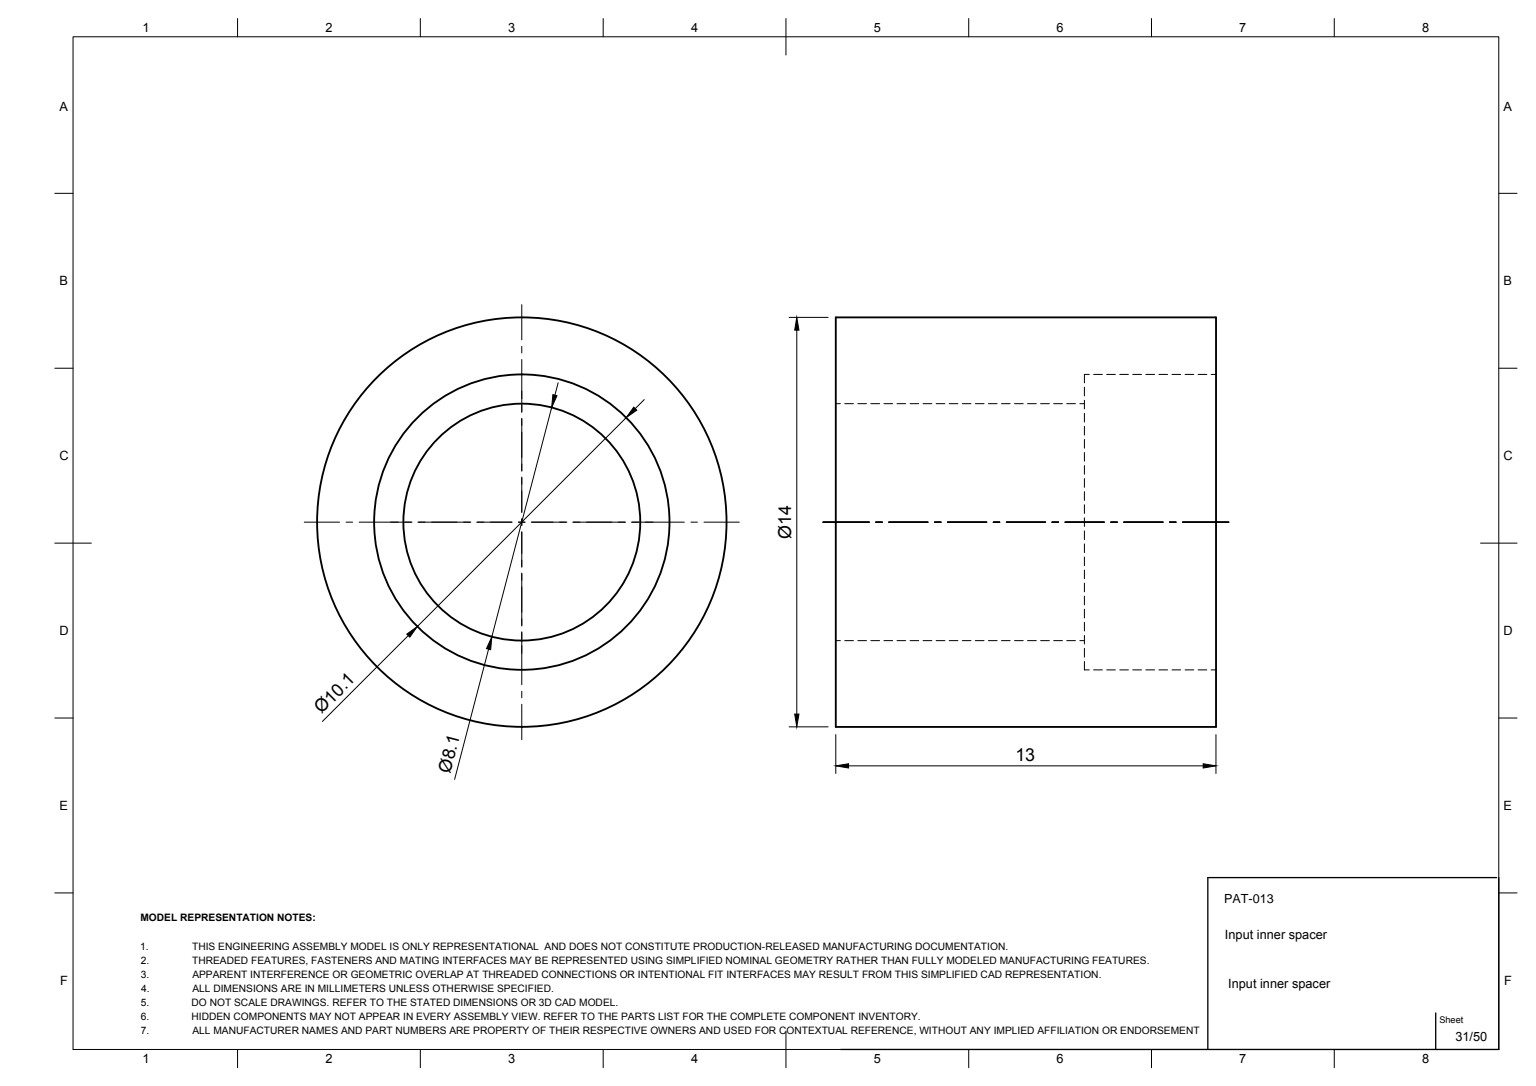
ISO-10303-21;
HEADER;
/* Generated by software containing ST-Developer
 * from STEP Tools, Inc. (www.steptools.com) 
 */

FILE_DESCRIPTION(
/* description */ ('Belt-driven linear axis on 2020 extrusion'),
/* implementation_level */ '2;1');

FILE_NAME(
/* name */ 'Input inner spacer.step',
/* time_stamp */ '2026-10-28T03:26:09-07:00',
/* author */ (''),
/* organization */ (''),
/* preprocessor_version */ 'ST-DEVELOPER v20.2',
/* originating_system */ 'Autodesk Translation Framework v15.17.0.0',
/* authorisation */ '');

FILE_SCHEMA (('AUTOMOTIVE_DESIGN { 1 0 10303 214 3 1 1 }'));
ENDSEC;

DATA;
#10=MECHANICAL_DESIGN_GEOMETRIC_PRESENTATION_REPRESENTATION('',(#644),#20096);
#542=SHAPE_REPRESENTATION_RELATIONSHIP('SRR','None',#20340,#588);
#588=ADVANCED_BREP_SHAPE_REPRESENTATION('',(#699),#20071);
#644=STYLED_ITEM('',(#20664),#699);
#699=MANIFOLD_SOLID_BREP('Body1',#10958);
#833=FACE_BOUND('',#2368,.T.);
#834=FACE_BOUND('',#2372,.T.);
#835=FACE_BOUND('',#2374,.T.);
#1116=PLANE('',#12215);
#1117=PLANE('',#12222);
#1118=PLANE('',#12223);
#1629=FACE_OUTER_BOUND('',#2366,.T.);
#1630=FACE_OUTER_BOUND('',#2367,.T.);
#1631=FACE_OUTER_BOUND('',#2369,.T.);
#1632=FACE_OUTER_BOUND('',#2370,.T.);
#1633=FACE_OUTER_BOUND('',#2371,.T.);
#1634=FACE_OUTER_BOUND('',#2373,.T.);
#2366=EDGE_LOOP('',(#8995,#8996,#8997,#8998));
#2367=EDGE_LOOP('',(#8999));
#2368=EDGE_LOOP('',(#9000));
#2369=EDGE_LOOP('',(#9001,#9002,#9003,#9004));
#2370=EDGE_LOOP('',(#9005,#9006,#9007,#9008));
#2371=EDGE_LOOP('',(#9009));
#2372=EDGE_LOOP('',(#9010));
#2373=EDGE_LOOP('',(#9011));
#2374=EDGE_LOOP('',(#9012));
#3209=LINE('',#18447,#4066);
#3210=LINE('',#18454,#4067);
#3211=LINE('',#18460,#4068);
#4066=VECTOR('',#14777,0.505);
#4067=VECTOR('',#14786,0.405);
#4068=VECTOR('',#14793,0.7);
#4686=CIRCLE('',#12213,0.505);
#4687=CIRCLE('',#12214,0.505);
#4688=CIRCLE('',#12216,0.405);
#4689=CIRCLE('',#12218,0.405);
#4690=CIRCLE('',#12220,0.7);
#4691=CIRCLE('',#12221,0.7);
#5481=VERTEX_POINT('',#18444);
#5482=VERTEX_POINT('',#18446);
#5483=VERTEX_POINT('',#18450);
#5484=VERTEX_POINT('',#18453);
#5485=VERTEX_POINT('',#18457);
#5486=VERTEX_POINT('',#18459);
#6712=EDGE_CURVE('',#5481,#5481,#4686,.T.);
#6713=EDGE_CURVE('',#5481,#5482,#3209,.T.);
#6714=EDGE_CURVE('',#5482,#5482,#4687,.T.);
#6715=EDGE_CURVE('',#5483,#5483,#4688,.T.);
#6716=EDGE_CURVE('',#5483,#5484,#3210,.T.);
#6717=EDGE_CURVE('',#5484,#5484,#4689,.T.);
#6718=EDGE_CURVE('',#5485,#5485,#4690,.T.);
#6719=EDGE_CURVE('',#5485,#5486,#3211,.T.);
#6720=EDGE_CURVE('',#5486,#5486,#4691,.T.);
#8995=ORIENTED_EDGE('',*,*,#6712,.F.);
#8996=ORIENTED_EDGE('',*,*,#6713,.T.);
#8997=ORIENTED_EDGE('',*,*,#6714,.F.);
#8998=ORIENTED_EDGE('',*,*,#6713,.F.);
#8999=ORIENTED_EDGE('',*,*,#6712,.T.);
#9000=ORIENTED_EDGE('',*,*,#6715,.F.);
#9001=ORIENTED_EDGE('',*,*,#6715,.T.);
#9002=ORIENTED_EDGE('',*,*,#6716,.T.);
#9003=ORIENTED_EDGE('',*,*,#6717,.T.);
#9004=ORIENTED_EDGE('',*,*,#6716,.F.);
#9005=ORIENTED_EDGE('',*,*,#6718,.F.);
#9006=ORIENTED_EDGE('',*,*,#6719,.T.);
#9007=ORIENTED_EDGE('',*,*,#6720,.T.);
#9008=ORIENTED_EDGE('',*,*,#6719,.F.);
#9009=ORIENTED_EDGE('',*,*,#6718,.T.);
#9010=ORIENTED_EDGE('',*,*,#6714,.T.);
#9011=ORIENTED_EDGE('',*,*,#6720,.F.);
#9012=ORIENTED_EDGE('',*,*,#6717,.F.);
#10204=CYLINDRICAL_SURFACE('',#12212,0.505);
#10205=CYLINDRICAL_SURFACE('',#12217,0.405);
#10206=CYLINDRICAL_SURFACE('',#12219,0.7);
#10680=ADVANCED_FACE('',(#1629),#10204,.F.);
#10681=ADVANCED_FACE('',(#1630,#833),#1116,.T.);
#10682=ADVANCED_FACE('',(#1631),#10205,.F.);
#10683=ADVANCED_FACE('',(#1632),#10206,.T.);
#10684=ADVANCED_FACE('',(#1633,#834),#1117,.T.);
#10685=ADVANCED_FACE('',(#1634,#835),#1118,.F.);
#10958=CLOSED_SHELL('',(#10680,#10681,#10682,#10683,#10684,#10685));
#12211=AXIS2_PLACEMENT_3D('',#18442,#14771,#14772);
#12212=AXIS2_PLACEMENT_3D('',#18443,#14773,#14774);
#12213=AXIS2_PLACEMENT_3D('',#18445,#14775,#14776);
#12214=AXIS2_PLACEMENT_3D('',#18448,#14778,#14779);
#12215=AXIS2_PLACEMENT_3D('',#18449,#14780,#14781);
#12216=AXIS2_PLACEMENT_3D('',#18451,#14782,#14783);
#12217=AXIS2_PLACEMENT_3D('',#18452,#14784,#14785);
#12218=AXIS2_PLACEMENT_3D('',#18455,#14787,#14788);
#12219=AXIS2_PLACEMENT_3D('',#18456,#14789,#14790);
#12220=AXIS2_PLACEMENT_3D('',#18458,#14791,#14792);
#12221=AXIS2_PLACEMENT_3D('',#18461,#14794,#14795);
#12222=AXIS2_PLACEMENT_3D('',#18462,#14796,#14797);
#12223=AXIS2_PLACEMENT_3D('',#18463,#14798,#14799);
#14771=DIRECTION('axis',(0.,0.,1.));
#14772=DIRECTION('refdir',(1.,0.,0.));
#14773=DIRECTION('center_axis',(0.,1.,0.));
#14774=DIRECTION('ref_axis',(1.,0.,0.));
#14775=DIRECTION('center_axis',(0.,1.,0.));
#14776=DIRECTION('ref_axis',(1.,0.,0.));
#14777=DIRECTION('',(0.,1.,0.));
#14778=DIRECTION('center_axis',(0.,-1.,0.));
#14779=DIRECTION('ref_axis',(1.,0.,0.));
#14780=DIRECTION('center_axis',(0.,1.,0.));
#14781=DIRECTION('ref_axis',(1.,0.,0.));
#14782=DIRECTION('center_axis',(0.,1.,0.));
#14783=DIRECTION('ref_axis',(1.,0.,0.));
#14784=DIRECTION('center_axis',(0.,1.,0.));
#14785=DIRECTION('ref_axis',(1.,0.,0.));
#14786=DIRECTION('',(0.,-1.,0.));
#14787=DIRECTION('center_axis',(0.,-1.,0.));
#14788=DIRECTION('ref_axis',(1.,0.,0.));
#14789=DIRECTION('center_axis',(0.,1.,0.));
#14790=DIRECTION('ref_axis',(1.,0.,0.));
#14791=DIRECTION('center_axis',(0.,1.,0.));
#14792=DIRECTION('ref_axis',(1.,0.,0.));
#14793=DIRECTION('',(0.,-1.,0.));
#14794=DIRECTION('center_axis',(0.,1.,0.));
#14795=DIRECTION('ref_axis',(1.,0.,0.));
#14796=DIRECTION('center_axis',(0.,1.,0.));
#14797=DIRECTION('ref_axis',(1.,0.,0.));
#14798=DIRECTION('center_axis',(0.,1.,0.));
#14799=DIRECTION('ref_axis',(1.,0.,0.));
#18442=CARTESIAN_POINT('',(0.,0.,0.));
#18443=CARTESIAN_POINT('Origin',(0.,-1.8,7.));
#18444=CARTESIAN_POINT('',(-0.505,-1.8,7.));
#18445=CARTESIAN_POINT('Origin',(0.,-1.8,7.));
#18446=CARTESIAN_POINT('',(-0.505,-1.35,7.));
#18447=CARTESIAN_POINT('',(-0.505,-1.8,7.));
#18448=CARTESIAN_POINT('Origin',(0.,-1.35,7.));
#18449=CARTESIAN_POINT('Origin',(0.,-1.8,7.));
#18450=CARTESIAN_POINT('',(-0.405,-1.8,7.));
#18451=CARTESIAN_POINT('Origin',(0.,-1.8,7.));
#18452=CARTESIAN_POINT('Origin',(0.,-2.65,7.));
#18453=CARTESIAN_POINT('',(-0.405,-2.65,7.));
#18454=CARTESIAN_POINT('',(-0.405,-2.65,7.));
#18455=CARTESIAN_POINT('Origin',(0.,-2.65,7.));
#18456=CARTESIAN_POINT('Origin',(0.,-2.65,7.));
#18457=CARTESIAN_POINT('',(-0.7,-1.35,7.));
#18458=CARTESIAN_POINT('Origin',(0.,-1.35,7.));
#18459=CARTESIAN_POINT('',(-0.7,-2.65,7.));
#18460=CARTESIAN_POINT('',(-0.7,-2.65,7.));
#18461=CARTESIAN_POINT('Origin',(0.,-2.65,7.));
#18462=CARTESIAN_POINT('Origin',(0.,-1.35,7.));
#18463=CARTESIAN_POINT('Origin',(0.,-2.65,7.));
#20017=UNCERTAINTY_MEASURE_WITH_UNIT(LENGTH_MEASURE(0.001),#20097,
'DISTANCE_ACCURACY_VALUE',
'Maximum model space distance between geometric entities at asserted c
onnectivities');
#20042=UNCERTAINTY_MEASURE_WITH_UNIT(LENGTH_MEASURE(0.001),#20097,
'DISTANCE_ACCURACY_VALUE',
'Maximum model space distance between geometric entities at asserted c
onnectivities');
#20071=(
GEOMETRIC_REPRESENTATION_CONTEXT(3)
GLOBAL_UNCERTAINTY_ASSIGNED_CONTEXT((#20017))
GLOBAL_UNIT_ASSIGNED_CONTEXT((#20097,#20099,#20100))
REPRESENTATION_CONTEXT('','3D')
);
#20096=(
GEOMETRIC_REPRESENTATION_CONTEXT(3)
GLOBAL_UNCERTAINTY_ASSIGNED_CONTEXT((#20042))
GLOBAL_UNIT_ASSIGNED_CONTEXT((#20097,#20099,#20100))
REPRESENTATION_CONTEXT('','3D')
);
#20097=(
LENGTH_UNIT()
NAMED_UNIT(*)
SI_UNIT(.CENTI.,.METRE.)
);
#20099=(
NAMED_UNIT(*)
PLANE_ANGLE_UNIT()
SI_UNIT($,.RADIAN.)
);
#20100=(
NAMED_UNIT(*)
SI_UNIT($,.STERADIAN.)
SOLID_ANGLE_UNIT()
);
#20129=SHAPE_DEFINITION_REPRESENTATION(#20187,#20340);
#20187=PRODUCT_DEFINITION_SHAPE('',$,#20394);
#20340=SHAPE_REPRESENTATION('',(#12211),#20071);
#20365=PRODUCT_DEFINITION_CONTEXT('part definition',#20526,'design');
#20394=PRODUCT_DEFINITION('Input inner spacer','Input inner spacer',#20447,
#20365);
#20447=PRODUCT_DEFINITION_FORMATION('',$,#20556);
#20526=APPLICATION_CONTEXT(
'Core Data for Automotive Mechanical Design Process');
#20527=PRODUCT_CONTEXT('part definition',#20526,'mechanical');
#20556=PRODUCT('Input inner spacer','Input inner spacer',
'Input inner spacer',(#20527));
#20658=COLOUR_RGB('Off White',0.89,0.88,0.83);
#20659=FILL_AREA_STYLE_COLOUR('',#20658);
#20660=FILL_AREA_STYLE('',(#20659));
#20661=SURFACE_STYLE_FILL_AREA(#20660);
#20662=SURFACE_SIDE_STYLE('',(#20661));
#20663=SURFACE_STYLE_USAGE(.BOTH.,#20662);
#20664=PRESENTATION_STYLE_ASSIGNMENT((#20663));
ENDSEC;
END-ISO-10303-21;
